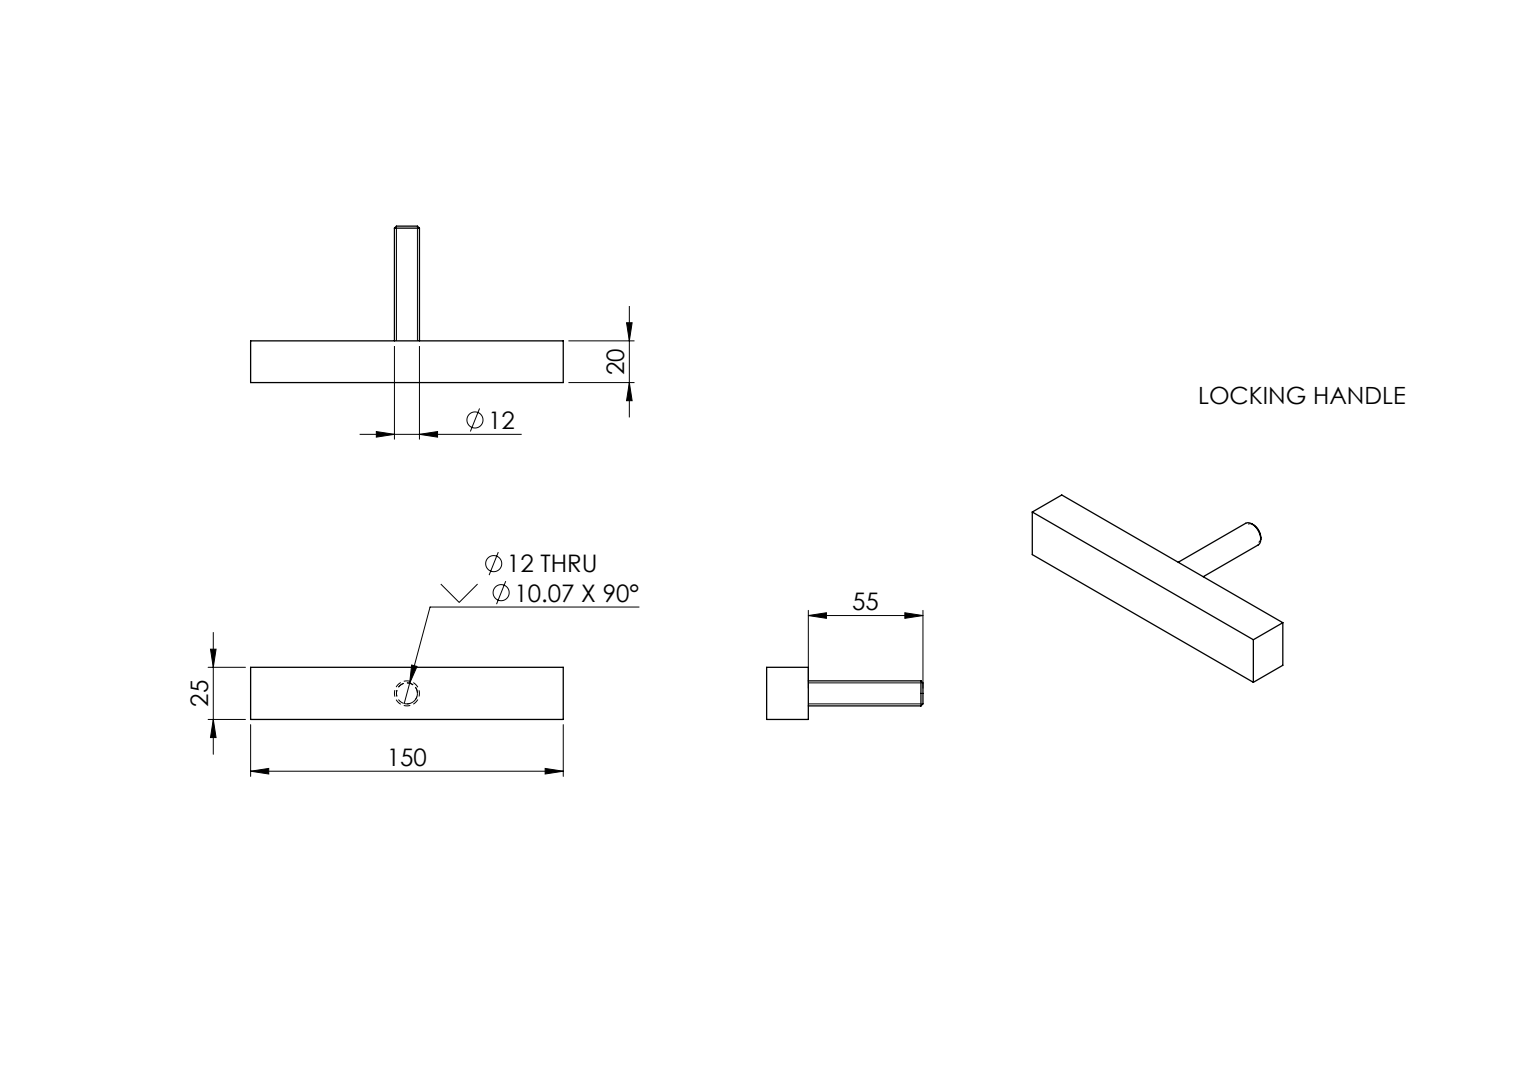
ISO-10303-21;
HEADER;
FILE_DESCRIPTION (('STEP AP214'),
    '1' );
FILE_NAME ('Locking handle.step',
    '2026-10-22T16:49:52',
    ( '' ),
    ( '' ),
    'SwSTEP 2.0',
    'SolidWorks 2026',
    '' );
FILE_SCHEMA (( 'AUTOMOTIVE_DESIGN' ));
ENDSEC;

DATA;
#11=EDGE_CURVE ( 'NONE', #3738, #432, #4098, .T. ) ;
#12=ORIENTED_EDGE ( 'NONE', *, *, #4828, .T. ) ;
#13=DIRECTION ( 'NONE',  ( 7.401486830834378251E-16, -1.000000000000000000, 0.000000000000000000 ) ) ;
#16=EDGE_CURVE ( 'NONE', #5260, #261, #3181, .T. ) ;
#28=EDGE_LOOP ( 'NONE', ( #1037, #4864, #2855, #4479 ) ) ;
#37=CARTESIAN_POINT ( 'NONE',  ( -74.99999999999998579, 610.0000000000000000, 49.99999999999998579 ) ) ;
#52=EDGE_CURVE ( 'NONE', #4486, #4891, #4610, .T. ) ;
#53=EDGE_LOOP ( 'NONE', ( #12, #4860, #912, #4381 ) ) ;
#54=AXIS2_PLACEMENT_3D ( 'NONE', #1971, #1612, #2923 ) ;
#85=FACE_OUTER_BOUND ( 'NONE', #3426, .T. ) ;
#114=DIRECTION ( 'NONE',  ( 1.000000000000000000, 0.000000000000000000, 0.000000000000000000 ) ) ;
#120=EDGE_LOOP ( 'NONE', ( #3988, #3057, #2483, #2092 ) ) ;
#121=SHAPE_REPRESENTATION ( 'Locking handle', ( #4154 ), #2227 ) ;
#140=AXIS2_PLACEMENT_3D ( 'NONE', #4031, #279, #2385 ) ;
#141=COLOUR_RGB ( '',0.8941176470588234615, 0.8941176470588234615, 0.8941176470588234615 ) ;
#146=CARTESIAN_POINT ( 'NONE',  ( -74.99999999999998579, 582.4999999999997726, 49.99999999999998579 ) ) ;
#172=MECHANICAL_DESIGN_GEOMETRIC_PRESENTATION_REPRESENTATION('',(#4869),#4866);
#231=PLANE ( 'NONE',  #3894 ) ;
#258=MANIFOLD_SOLID_BREP ( 'M12 Machine Threads Stud1', #3451 ) ;
#259=ORIENTED_EDGE ( 'NONE', *, *, #2872, .T. ) ;
#261=VERTEX_POINT ( 'NONE', #1126 ) ;
#275=DIRECTION ( 'NONE',  ( 1.000000000000000000, 0.000000000000000000, 0.000000000000000000 ) ) ;
#276=ORIENTED_EDGE ( 'NONE', *, *, #1791, .T. ) ;
#279=DIRECTION ( 'NONE',  ( -0.000000000000000000, -0.000000000000000000, 1.000000000000000000 ) ) ;
#283=DIRECTION ( 'NONE',  ( -0.000000000000000000, -0.000000000000000000, 1.000000000000000000 ) ) ;
#295=AXIS2_PLACEMENT_3D ( 'NONE', #2964, #518, #4278 ) ;
#317=PLANE ( 'NONE',  #5199 ) ;
#334=AXIS2_PLACEMENT_3D ( 'NONE', #394, #283, #1936 ) ;
#343=ORIENTED_EDGE ( 'NONE', *, *, #2742, .T. ) ;
#349=CARTESIAN_POINT ( 'NONE',  ( -1.144917494144692998E-14, 570.0000000000000000, -24.99999999999998579 ) ) ;
#372=ADVANCED_FACE ( 'NONE', ( #4132 ), #2916, .F. ) ;
#373=ORIENTED_EDGE ( 'NONE', *, *, #3431, .F. ) ;
#388=PLANE ( 'NONE',  #3538 ) ;
#390=VECTOR ( 'NONE', #4500, 1000.000000000000000 ) ;
#394=CARTESIAN_POINT ( 'NONE',  ( -1.144917494144692998E-14, 570.0000000000000000, -24.03599999999999071 ) ) ;
#409=ORIENTED_EDGE ( 'NONE', *, *, #3431, .T. ) ;
#432=VERTEX_POINT ( 'NONE', #439 ) ;
#439=CARTESIAN_POINT ( 'NONE',  ( -74.99999999999998579, 582.4999999999997726, 49.99999999999998579 ) ) ;
#458=EDGE_CURVE ( 'NONE', #3578, #4918, #3803, .T. ) ;
#469=SURFACE_STYLE_USAGE ( .BOTH. , #4208 ) ;
#470=EDGE_CURVE ( 'NONE', #4891, #4946, #540, .T. ) ;
#501=APPLICATION_CONTEXT ( 'automotive_design' ) ;
#510=DIRECTION ( 'NONE',  ( -0.000000000000000000, -0.000000000000000000, 1.000000000000000000 ) ) ;
#518=DIRECTION ( 'NONE',  ( 0.000000000000000000, 0.000000000000000000, -1.000000000000000000 ) ) ;
#533=EDGE_CURVE ( 'NONE', #432, #3578, #4203, .T. ) ;
#540=LINE ( 'NONE', #569, #3063 ) ;
#569=CARTESIAN_POINT ( 'NONE',  ( 1.410908427127813464E-14, 582.4999999999997726, 30.00000000000000711 ) ) ;
#581=LINE ( 'NONE', #1466, #1103 ) ;
#594=ORIENTED_EDGE ( 'NONE', *, *, #829, .T. ) ;
#600=DIRECTION ( 'NONE',  ( -0.000000000000000000, -0.000000000000000000, 1.000000000000000000 ) ) ;
#608=ORIENTED_EDGE ( 'NONE', *, *, #458, .F. ) ;
#671=ORIENTED_EDGE ( 'NONE', *, *, #1136, .T. ) ;
#679=AXIS2_PLACEMENT_3D ( 'NONE', #2078, #13, #3676 ) ;
#688=EDGE_CURVE ( 'NONE', #1702, #1418, #2388, .T. ) ;
#729=CARTESIAN_POINT ( 'NONE',  ( 75.00000000000001421, 610.0000000000000000, 30.00000000000002487 ) ) ;
#757=UNCERTAINTY_MEASURE_WITH_UNIT (LENGTH_MEASURE( 1.000000000000000082E-05 ), #1560, 'distance_accuracy_value', 'NONE');
#760=ADVANCED_FACE ( 'NONE', ( #5235 ), #3158, .T. ) ;
#764=ORIENTED_EDGE ( 'NONE', *, *, #1472, .T. ) ;
#769=DIRECTION ( 'NONE',  ( 1.000000000000000000, 0.000000000000000000, 0.000000000000000000 ) ) ;
#805=ORIENTED_EDGE ( 'NONE', *, *, #4792, .T. ) ;
#812=CARTESIAN_POINT ( 'NONE',  ( -1.144917494144692998E-14, 570.0000000000000000, 30.00000000000001066 ) ) ;
#829=EDGE_CURVE ( 'NONE', #3578, #1196, #3313, .T. ) ;
#830=LINE ( 'NONE', #3422, #4489 ) ;
#839=AXIS2_PLACEMENT_3D ( 'NONE', #349, #4430, #864 ) ;
#864=DIRECTION ( 'NONE',  ( 1.000000000000000000, 0.000000000000000000, 0.000000000000000000 ) ) ;
#884=CARTESIAN_POINT ( 'NONE',  ( 5.999999999999983125, 570.0000000000000000, -24.03599999999999071 ) ) ;
#907=CARTESIAN_POINT ( 'NONE',  ( -1.144917494144692998E-14, 570.0000000000000000, 30.00000000000001066 ) ) ;
#909=AXIS2_PLACEMENT_3D ( 'NONE', #907, #510, #3839 ) ;
#912=ORIENTED_EDGE ( 'NONE', *, *, #533, .F. ) ;
#926=DIRECTION ( 'NONE',  ( 1.000000000000000000, 0.000000000000000000, -0.000000000000000000 ) ) ;
#953=CARTESIAN_POINT ( 'NONE',  ( 75.00000000000001421, 610.0000000000000000, 50.00000000000002132 ) ) ;
#965=VECTOR ( 'NONE', #2398, 1000.000000000000000 ) ;
#999=VECTOR ( 'NONE', #3243, 1000.000000000000000 ) ;
#1010=VECTOR ( 'NONE', #1523, 999.9999999999998863 ) ;
#1013=EDGE_LOOP ( 'NONE', ( #4222, #3217 ) ) ;
#1015=CARTESIAN_POINT ( 'NONE',  ( -1.144917494144692998E-14, 570.0000000000000000, -24.03599999999999071 ) ) ;
#1019=DIRECTION ( 'NONE',  ( -0.000000000000000000, -0.000000000000000000, -1.000000000000000000 ) ) ;
#1036=ORIENTED_EDGE ( 'NONE', *, *, #3071, .T. ) ;
#1037=ORIENTED_EDGE ( 'NONE', *, *, #2742, .F. ) ;
#1048=LINE ( 'NONE', #4368, #1525 ) ;
#1092=PRODUCT_DEFINITION_FORMATION_WITH_SPECIFIED_SOURCE ( 'ANY', '', #4530, .NOT_KNOWN. ) ;
#1103=VECTOR ( 'NONE', #2269, 999.9999999999998863 ) ;
#1126=CARTESIAN_POINT ( 'NONE',  ( -5.036000000000011134, 570.0000000000000000, -24.99999999999998579 ) ) ;
#1134=( NAMED_UNIT ( * ) SI_UNIT ( $, .STERADIAN. ) SOLID_ANGLE_UNIT ( ) );
#1136=EDGE_CURVE ( 'NONE', #2556, #2061, #2486, .T. ) ;
#1149=CARTESIAN_POINT ( 'NONE',  ( 75.00000000000000000, 582.4999999999997726, 50.00000000000001421 ) ) ;
#1153=DIRECTION ( 'NONE',  ( -2.081668171172168513E-16, 0.000000000000000000, 1.000000000000000000 ) ) ;
#1196=VERTEX_POINT ( 'NONE', #1862 ) ;
#1223=DIRECTION ( 'NONE',  ( 0.000000000000000000, 0.000000000000000000, 1.000000000000000000 ) ) ;
#1236=CARTESIAN_POINT ( 'NONE',  ( 5.999999999999988454, 570.0000000000000000, 30.00000000000001066 ) ) ;
#1242=PLANE ( 'NONE',  #54 ) ;
#1259=LINE ( 'NONE', #3374, #1983 ) ;
#1260=SHAPE_REPRESENTATION_RELATIONSHIP ( 'NONE' , 'NONE' ,  #121, #2208 ) ;
#1261=CONICAL_SURFACE ( 'NONE', #5087, 5.999999999999993783, 0.7853981633974491672 ) ;
#1300=ADVANCED_FACE ( 'NONE', ( #4202 ), #3875, .T. ) ;
#1308=DIRECTION ( 'NONE',  ( 1.000000000000000000, -0.000000000000000000, 2.081668171172168513E-16 ) ) ;
#1314=ORIENTED_EDGE ( 'NONE', *, *, #1686, .T. ) ;
#1318=FACE_OUTER_BOUND ( 'NONE', #4015, .T. ) ;
#1329=DIRECTION ( 'NONE',  ( -0.000000000000000000, -0.000000000000000000, 1.000000000000000000 ) ) ;
#1353=CARTESIAN_POINT ( 'NONE',  ( 5.035999999999988042, 570.0000000000000000, -24.99999999999998579 ) ) ;
#1381=DIRECTION ( 'NONE',  ( 0.000000000000000000, -1.000000000000000000, 0.000000000000000000 ) ) ;
#1389=ORIENTED_EDGE ( 'NONE', *, *, #1472, .F. ) ;
#1402=CARTESIAN_POINT ( 'NONE',  ( 75.00000000000000000, 582.4999999999997726, 30.00000000000002132 ) ) ;
#1405=FACE_OUTER_BOUND ( 'NONE', #5287, .T. ) ;
#1418=VERTEX_POINT ( 'NONE', #3558 ) ;
#1431=CARTESIAN_POINT ( 'NONE',  ( 75.00000000000000000, 582.4999999999997726, 50.00000000000001421 ) ) ;
#1465=( LENGTH_UNIT ( ) NAMED_UNIT ( * ) SI_UNIT ( .MILLI., .METRE. ) );
#1466=CARTESIAN_POINT ( 'NONE',  ( -6.000000000000005329, 570.0000000000000000, -24.03599999999999071 ) ) ;
#1472=EDGE_CURVE ( 'NONE', #4918, #3738, #3088, .T. ) ;
#1504=CARTESIAN_POINT ( 'NONE',  ( 1.410908427127813464E-14, 582.4999999999997726, 50.00000000000000000 ) ) ;
#1512=DIRECTION ( 'NONE',  ( -0.000000000000000000, -0.000000000000000000, 1.000000000000000000 ) ) ;
#1523=DIRECTION ( 'NONE',  ( 0.7071067811865482389, 0.000000000000000000, 0.7071067811865469066 ) ) ;
#1525=VECTOR ( 'NONE', #2740, 1000.000000000000000 ) ;
#1527=ADVANCED_FACE ( 'NONE', ( #1405 ), #1261, .T. ) ;
#1531=CARTESIAN_POINT ( 'NONE',  ( -6.245004513516506329E-15, 557.4999999999997726, 50.00000000000000000 ) ) ;
#1552=CARTESIAN_POINT ( 'NONE',  ( -1.144917494144692998E-14, 570.0000000000000000, -24.03599999999999071 ) ) ;
#1553=( NAMED_UNIT ( * ) PLANE_ANGLE_UNIT ( ) SI_UNIT ( $, .RADIAN. ) );
#1555=FACE_BOUND ( 'NONE', #1013, .T. ) ;
#1560=( LENGTH_UNIT ( ) NAMED_UNIT ( * ) SI_UNIT ( .MILLI., .METRE. ) );
#1580=EDGE_CURVE ( 'NONE', #3738, #4891, #4131, .T. ) ;
#1612=DIRECTION ( 'NONE',  ( -1.000000000000000000, 5.551115123125753120E-16, 0.000000000000000000 ) ) ;
#1647=FACE_OUTER_BOUND ( 'NONE', #3306, .T. ) ;
#1686=EDGE_CURVE ( 'NONE', #2061, #2556, #4819, .T. ) ;
#1693=SURFACE_STYLE_FILL_AREA ( #3663 ) ;
#1702=VERTEX_POINT ( 'NONE', #1236 ) ;
#1787=( GEOMETRIC_REPRESENTATION_CONTEXT ( 3 ) GLOBAL_UNCERTAINTY_ASSIGNED_CONTEXT ( ( #4190 ) ) GLOBAL_UNIT_ASSIGNED_CONTEXT ( ( #3858, #4097, #4997 ) ) REPRESENTATION_CONTEXT ( 'NONE', 'WORKASPACE' ) );
#1791=EDGE_CURVE ( 'NONE', #2061, #1418, #3073, .T. ) ;
#1844=CARTESIAN_POINT ( 'NONE',  ( 74.99999999999998579, 557.4999999999997726, 50.00000000000002132 ) ) ;
#1862=CARTESIAN_POINT ( 'NONE',  ( -74.99999999999998579, 557.4999999999997726, 29.99999999999999289 ) ) ;
#1910=CARTESIAN_POINT ( 'NONE',  ( 74.99999999999998579, 557.4999999999997726, 30.00000000000002487 ) ) ;
#1923=CARTESIAN_POINT ( 'NONE',  ( -1.144917494144692998E-14, 570.0000000000000000, 30.00000000000001066 ) ) ;
#1936=DIRECTION ( 'NONE',  ( 1.000000000000000000, 0.000000000000000000, 0.000000000000000000 ) ) ;
#1963=( NAMED_UNIT ( * ) SI_UNIT ( $, .STERADIAN. ) SOLID_ANGLE_UNIT ( ) );
#1971=CARTESIAN_POINT ( 'NONE',  ( 75.00000000000001421, 610.0000000000000000, 50.00000000000002132 ) ) ;
#1972=DIRECTION ( 'NONE',  ( 0.000000000000000000, 1.000000000000000000, -0.000000000000000000 ) ) ;
#1983=VECTOR ( 'NONE', #4207, 1000.000000000000000 ) ;
#2022=CARTESIAN_POINT ( 'NONE',  ( -6.245004513516507118E-15, 0.000000000000000000, 30.00000000000001066 ) ) ;
#2032=VECTOR ( 'NONE', #4152, 1000.000000000000000 ) ;
#2057=CIRCLE ( 'NONE', #140, 5.035999999999999588 ) ;
#2061=VERTEX_POINT ( 'NONE', #4174 ) ;
#2068=AXIS2_PLACEMENT_3D ( 'NONE', #812, #4268, #114 ) ;
#2078=CARTESIAN_POINT ( 'NONE',  ( 1.410908427127813464E-14, 582.4999999999997726, 50.00000000000000000 ) ) ;
#2083=ORIENTED_EDGE ( 'NONE', *, *, #4792, .F. ) ;
#2092=ORIENTED_EDGE ( 'NONE', *, *, #1580, .T. ) ;
#2109=ORIENTED_EDGE ( 'NONE', *, *, #2872, .F. ) ;
#2113=AXIS2_PLACEMENT_3D ( 'NONE', #1923, #1512, #4872 ) ;
#2119=AXIS2_PLACEMENT_3D ( 'NONE', #5170, #3491, #2753 ) ;
#2135=ORIENTED_EDGE ( 'NONE', *, *, #52, .T. ) ;
#2163=EDGE_LOOP ( 'NONE', ( #671, #276, #2307, #5328 ) ) ;
#2188=PRODUCT_DEFINITION ( 'UNKNOWN', '', #1092, #5338 ) ;
#2203=DIRECTION ( 'NONE',  ( -1.000000000000000000, -7.401486830834378251E-16, -2.081668171172168513E-16 ) ) ;
#2206=CARTESIAN_POINT ( 'NONE',  ( -74.99999999999998579, 610.0000000000000000, 29.99999999999999289 ) ) ;
#2208=ADVANCED_BREP_SHAPE_REPRESENTATION ( '', ( #258, #4154 ), #2227 ) ;
#2216=LINE ( 'NONE', #146, #3281 ) ;
#2218=ADVANCED_FACE ( 'NONE', ( #1318 ), #4636, .T. ) ;
#2227=( GEOMETRIC_REPRESENTATION_CONTEXT ( 3 ) GLOBAL_UNCERTAINTY_ASSIGNED_CONTEXT ( ( #757 ) ) GLOBAL_UNIT_ASSIGNED_CONTEXT ( ( #1560, #4036, #1134 ) ) REPRESENTATION_CONTEXT ( 'NONE', 'WORKASPACE' ) );
#2229=VECTOR ( 'NONE', #3421, 1000.000000000000000 ) ;
#2258=ORIENTED_EDGE ( 'NONE', *, *, #1580, .F. ) ;
#2269=DIRECTION ( 'NONE',  ( -0.7071067811865482389, 8.659560562354941486E-17, 0.7071067811865469066 ) ) ;
#2307=ORIENTED_EDGE ( 'NONE', *, *, #688, .F. ) ;
#2373=DIRECTION ( 'NONE',  ( -0.000000000000000000, -0.000000000000000000, 1.000000000000000000 ) ) ;
#2385=DIRECTION ( 'NONE',  ( 1.000000000000000000, 0.000000000000000000, 0.000000000000000000 ) ) ;
#2388=CIRCLE ( 'NONE', #2564, 6.000000000000000000 ) ;
#2398=DIRECTION ( 'NONE',  ( 5.551115123125753120E-16, 1.000000000000000000, 1.155557966632335381E-31 ) ) ;
#2430=VECTOR ( 'NONE', #1381, 1000.000000000000000 ) ;
#2434=CARTESIAN_POINT ( 'NONE',  ( 0.000000000000000000, 0.000000000000000000, 0.000000000000000000 ) ) ;
#2437=ADVANCED_FACE ( 'NONE', ( #3660 ), #1242, .F. ) ;
#2483=ORIENTED_EDGE ( 'NONE', *, *, #11, .F. ) ;
#2486=CIRCLE ( 'NONE', #2119, 5.999999999999993783 ) ;
#2550=CARTESIAN_POINT ( 'NONE',  ( -6.245004513516506329E-15, 557.4999999999997726, 50.00000000000000000 ) ) ;
#2556=VERTEX_POINT ( 'NONE', #884 ) ;
#2564=AXIS2_PLACEMENT_3D ( 'NONE', #4336, #2373, #4438 ) ;
#2589=PRODUCT_DEFINITION_SHAPE ( 'NONE', 'NONE',  #2188 ) ;
#2608=DIRECTION ( 'NONE',  ( -0.000000000000000000, 0.000000000000000000, -1.000000000000000000 ) ) ;
#2613=EDGE_CURVE ( 'NONE', #432, #4946, #2216, .T. ) ;
#2640=DIRECTION ( 'NONE',  ( -0.000000000000000000, -0.000000000000000000, 1.000000000000000000 ) ) ;
#2661=AXIS2_PLACEMENT_3D ( 'NONE', #1552, #2854, #4938 ) ;
#2740=DIRECTION ( 'NONE',  ( 1.000000000000000000, -0.000000000000000000, 2.081668171172168513E-16 ) ) ;
#2742=EDGE_CURVE ( 'NONE', #1196, #4486, #1048, .T. ) ;
#2753=DIRECTION ( 'NONE',  ( 1.000000000000000000, 0.000000000000000000, 0.000000000000000000 ) ) ;
#2765=PRODUCT_CONTEXT ( 'NONE', #501, 'mechanical' ) ;
#2833=ORIENTED_EDGE ( 'NONE', *, *, #11, .T. ) ;
#2838=VECTOR ( 'NONE', #2640, 1000.000000000000000 ) ;
#2847=EDGE_CURVE ( 'NONE', #261, #5260, #2057, .T. ) ;
#2854=DIRECTION ( 'NONE',  ( -0.000000000000000000, -0.000000000000000000, 1.000000000000000000 ) ) ;
#2855=ORIENTED_EDGE ( 'NONE', *, *, #470, .F. ) ;
#2858=DIRECTION ( 'NONE',  ( 1.000000000000000000, 0.000000000000000000, 2.081668171172168513E-16 ) ) ;
#2872=EDGE_CURVE ( 'NONE', #5260, #2556, #5275, .T. ) ;
#2878=ORIENTED_EDGE ( 'NONE', *, *, #1136, .F. ) ;
#2897=ADVANCED_FACE ( 'NONE', ( #1555, #5308 ), #388, .F. ) ;
#2916=PLANE ( 'NONE',  #679 ) ;
#2923=DIRECTION ( 'NONE',  ( -5.551115123125753120E-16, -1.000000000000000000, 0.000000000000000000 ) ) ;
#2964=CARTESIAN_POINT ( 'NONE',  ( 5.035999999999988042, 570.0000000000000000, -24.99999999999998579 ) ) ;
#2986=CARTESIAN_POINT ( 'NONE',  ( -74.99999999999998579, 610.0000000000000000, 49.99999999999998579 ) ) ;
#2992=PRESENTATION_STYLE_ASSIGNMENT (( #469 ) ) ;
#3057=ORIENTED_EDGE ( 'NONE', *, *, #2613, .F. ) ;
#3063=VECTOR ( 'NONE', #2203, 1000.000000000000000 ) ;
#3071=EDGE_CURVE ( 'NONE', #2556, #1702, #830, .T. ) ;
#3073=LINE ( 'NONE', #4691, #2838 ) ;
#3088=LINE ( 'NONE', #953, #4562 ) ;
#3120=DIRECTION ( 'NONE',  ( 5.551115123125753120E-16, 1.000000000000000000, 1.155557966632335381E-31 ) ) ;
#3158=CYLINDRICAL_SURFACE ( 'NONE', #2113, 5.999999999999996447 ) ;
#3181=CIRCLE ( 'NONE', #839, 5.035999999999999588 ) ;
#3217=ORIENTED_EDGE ( 'NONE', *, *, #4327, .T. ) ;
#3243=DIRECTION ( 'NONE',  ( -1.000000000000000000, -7.401486830834378251E-16, -2.081668171172168513E-16 ) ) ;
#3281=VECTOR ( 'NONE', #1019, 1000.000000000000000 ) ;
#3306=EDGE_LOOP ( 'NONE', ( #343, #2083, #608, #594 ) ) ;
#3313=LINE ( 'NONE', #5323, #2032 ) ;
#3374=CARTESIAN_POINT ( 'NONE',  ( 74.99999999999998579, 557.4999999999997726, 50.00000000000002132 ) ) ;
#3405=EDGE_LOOP ( 'NONE', ( #2135, #2258, #1389, #805 ) ) ;
#3421=DIRECTION ( 'NONE',  ( 0.000000000000000000, -1.000000000000000000, 0.000000000000000000 ) ) ;
#3422=CARTESIAN_POINT ( 'NONE',  ( 5.999999999999985789, 570.0000000000000000, 30.00000000000001066 ) ) ;
#3426=EDGE_LOOP ( 'NONE', ( #3604, #764, #2833, #4140 ) ) ;
#3431=EDGE_CURVE ( 'NONE', #261, #2061, #581, .T. ) ;
#3443=EDGE_LOOP ( 'NONE', ( #4424, #5015 ) ) ;
#3451=CLOSED_SHELL ( 'NONE', ( #760, #4270, #4206, #2437, #372, #4774, #4100, #2897, #1300, #1527, #2218 ) ) ;
#3491=DIRECTION ( 'NONE',  ( -0.000000000000000000, -0.000000000000000000, 1.000000000000000000 ) ) ;
#3500=ORIENTED_EDGE ( 'NONE', *, *, #16, .T. ) ;
#3522=CARTESIAN_POINT ( 'NONE',  ( -74.99999999999998579, 582.4999999999997726, 29.99999999999999289 ) ) ;
#3538=AXIS2_PLACEMENT_3D ( 'NONE', #2022, #1153, #2858 ) ;
#3558=CARTESIAN_POINT ( 'NONE',  ( -6.000000000000012434, 570.0000000000000000, 30.00000000000001066 ) ) ;
#3568=DIRECTION ( 'NONE',  ( -2.081668171172168513E-16, 0.000000000000000000, 1.000000000000000000 ) ) ;
#3578=VERTEX_POINT ( 'NONE', #5355 ) ;
#3604=ORIENTED_EDGE ( 'NONE', *, *, #458, .T. ) ;
#3624=FILL_AREA_STYLE_COLOUR ( '', #141 ) ;
#3660=FACE_OUTER_BOUND ( 'NONE', #3405, .T. ) ;
#3663=FILL_AREA_STYLE ('',( #3624 ) ) ;
#3676=DIRECTION ( 'NONE',  ( 1.000000000000000000, 7.401486830834378251E-16, 0.000000000000000000 ) ) ;
#3738=VERTEX_POINT ( 'NONE', #1431 ) ;
#3803=LINE ( 'NONE', #2550, #4513 ) ;
#3805=PLANE ( 'NONE',  #4593 ) ;
#3839=DIRECTION ( 'NONE',  ( 1.000000000000000000, 0.000000000000000000, 0.000000000000000000 ) ) ;
#3858=( LENGTH_UNIT ( ) NAMED_UNIT ( * ) SI_UNIT ( .MILLI., .METRE. ) );
#3875=PLANE ( 'NONE',  #295 ) ;
#3894=AXIS2_PLACEMENT_3D ( 'NONE', #5222, #3568, #5164 ) ;
#3908=LINE ( 'NONE', #2206, #2430 ) ;
#3983=ORIENTED_EDGE ( 'NONE', *, *, #2847, .T. ) ;
#3988=ORIENTED_EDGE ( 'NONE', *, *, #470, .T. ) ;
#4015=EDGE_LOOP ( 'NONE', ( #5372, #1314, #1036, #4748 ) ) ;
#4031=CARTESIAN_POINT ( 'NONE',  ( -1.144917494144692998E-14, 570.0000000000000000, -24.99999999999998579 ) ) ;
#4036=( NAMED_UNIT ( * ) PLANE_ANGLE_UNIT ( ) SI_UNIT ( $, .RADIAN. ) );
#4097=( NAMED_UNIT ( * ) PLANE_ANGLE_UNIT ( ) SI_UNIT ( $, .RADIAN. ) );
#4098=LINE ( 'NONE', #1504, #999 ) ;
#4100=ADVANCED_FACE ( 'NONE', ( #85 ), #231, .T. ) ;
#4117=EDGE_LOOP ( 'NONE', ( #3500, #409, #2878, #2109 ) ) ;
#4131=LINE ( 'NONE', #1149, #390 ) ;
#4132=FACE_OUTER_BOUND ( 'NONE', #120, .T. ) ;
#4140=ORIENTED_EDGE ( 'NONE', *, *, #533, .T. ) ;
#4152=DIRECTION ( 'NONE',  ( -0.000000000000000000, -0.000000000000000000, -1.000000000000000000 ) ) ;
#4154=AXIS2_PLACEMENT_3D ( 'NONE', #2434, #5290, #769 ) ;
#4172=CIRCLE ( 'NONE', #2068, 6.000000000000000000 ) ;
#4174=CARTESIAN_POINT ( 'NONE',  ( -6.000000000000005329, 570.0000000000000000, -24.03599999999999071 ) ) ;
#4190=UNCERTAINTY_MEASURE_WITH_UNIT (LENGTH_MEASURE( 1.000000000000000082E-05 ), #3858, 'distance_accuracy_value', 'NONE');
#4202=FACE_OUTER_BOUND ( 'NONE', #3443, .T. ) ;
#4203=LINE ( 'NONE', #2986, #2229 ) ;
#4206=ADVANCED_FACE ( 'NONE', ( #1647 ), #317, .F. ) ;
#4207=DIRECTION ( 'NONE',  ( -0.000000000000000000, -0.000000000000000000, -1.000000000000000000 ) ) ;
#4208=SURFACE_SIDE_STYLE ('',( #1693 ) ) ;
#4222=ORIENTED_EDGE ( 'NONE', *, *, #688, .T. ) ;
#4268=DIRECTION ( 'NONE',  ( -0.000000000000000000, -0.000000000000000000, 1.000000000000000000 ) ) ;
#4270=ADVANCED_FACE ( 'NONE', ( #4890 ), #5114, .T. ) ;
#4278=DIRECTION ( 'NONE',  ( -1.000000000000000000, 0.000000000000000000, -0.000000000000000000 ) ) ;
#4327=EDGE_CURVE ( 'NONE', #1418, #1702, #4172, .T. ) ;
#4336=CARTESIAN_POINT ( 'NONE',  ( -1.144917494144692998E-14, 570.0000000000000000, 30.00000000000001066 ) ) ;
#4368=CARTESIAN_POINT ( 'NONE',  ( -6.245004513516506329E-15, 557.4999999999997726, 30.00000000000000711 ) ) ;
#4381=ORIENTED_EDGE ( 'NONE', *, *, #2613, .T. ) ;
#4424=ORIENTED_EDGE ( 'NONE', *, *, #16, .F. ) ;
#4430=DIRECTION ( 'NONE',  ( -0.000000000000000000, -0.000000000000000000, 1.000000000000000000 ) ) ;
#4438=DIRECTION ( 'NONE',  ( 1.000000000000000000, 0.000000000000000000, 0.000000000000000000 ) ) ;
#4442=UNCERTAINTY_MEASURE_WITH_UNIT (LENGTH_MEASURE( 1.000000000000000082E-05 ), #1465, 'distance_accuracy_value', 'NONE');
#4447=CARTESIAN_POINT ( 'NONE',  ( 5.999999999999983125, 570.0000000000000000, -24.03599999999999071 ) ) ;
#4479=ORIENTED_EDGE ( 'NONE', *, *, #52, .F. ) ;
#4486=VERTEX_POINT ( 'NONE', #1910 ) ;
#4489=VECTOR ( 'NONE', #1329, 1000.000000000000000 ) ;
#4500=DIRECTION ( 'NONE',  ( -0.000000000000000000, -0.000000000000000000, -1.000000000000000000 ) ) ;
#4513=VECTOR ( 'NONE', #1308, 1000.000000000000000 ) ;
#4523=SHAPE_DEFINITION_REPRESENTATION ( #2589, #121 ) ;
#4530=PRODUCT ( 'Locking handle', 'Locking handle', '', ( #2765 ) ) ;
#4562=VECTOR ( 'NONE', #3120, 1000.000000000000000 ) ;
#4593=AXIS2_PLACEMENT_3D ( 'NONE', #37, #926, #2608 ) ;
#4610=LINE ( 'NONE', #729, #965 ) ;
#4636=CYLINDRICAL_SURFACE ( 'NONE', #909, 5.999999999999996447 ) ;
#4653=FACE_OUTER_BOUND ( 'NONE', #53, .T. ) ;
#4669=ORIENTED_EDGE ( 'NONE', *, *, #1686, .F. ) ;
#4691=CARTESIAN_POINT ( 'NONE',  ( -6.000000000000007994, 570.0000000000000000, 30.00000000000001066 ) ) ;
#4748=ORIENTED_EDGE ( 'NONE', *, *, #4327, .F. ) ;
#4774=ADVANCED_FACE ( 'NONE', ( #4653 ), #3805, .F. ) ;
#4792=EDGE_CURVE ( 'NONE', #4918, #4486, #1259, .T. ) ;
#4819=CIRCLE ( 'NONE', #2661, 5.999999999999993783 ) ;
#4828=EDGE_CURVE ( 'NONE', #4946, #1196, #3908, .T. ) ;
#4842=APPLICATION_CONTEXT ( 'automotive_design' ) ;
#4860=ORIENTED_EDGE ( 'NONE', *, *, #829, .F. ) ;
#4864=ORIENTED_EDGE ( 'NONE', *, *, #4828, .F. ) ;
#4866=( GEOMETRIC_REPRESENTATION_CONTEXT ( 3 ) GLOBAL_UNCERTAINTY_ASSIGNED_CONTEXT ( ( #4442 ) ) GLOBAL_UNIT_ASSIGNED_CONTEXT ( ( #1465, #1553, #1963 ) ) REPRESENTATION_CONTEXT ( 'NONE', 'WORKASPACE' ) );
#4869=STYLED_ITEM('',(#5440),#258);
#4872=DIRECTION ( 'NONE',  ( 1.000000000000000000, 0.000000000000000000, 0.000000000000000000 ) ) ;
#4890=FACE_OUTER_BOUND ( 'NONE', #4117, .T. ) ;
#4891=VERTEX_POINT ( 'NONE', #1402 ) ;
#4918=VERTEX_POINT ( 'NONE', #1844 ) ;
#4938=DIRECTION ( 'NONE',  ( 1.000000000000000000, 0.000000000000000000, 0.000000000000000000 ) ) ;
#4946=VERTEX_POINT ( 'NONE', #3522 ) ;
#4997=( NAMED_UNIT ( * ) SI_UNIT ( $, .STERADIAN. ) SOLID_ANGLE_UNIT ( ) );
#5015=ORIENTED_EDGE ( 'NONE', *, *, #2847, .F. ) ;
#5019=STYLED_ITEM ( 'NONE', ( #2992 ), #2208 ) ;
#5087=AXIS2_PLACEMENT_3D ( 'NONE', #1015, #600, #275 ) ;
#5114=CONICAL_SURFACE ( 'NONE', #334, 5.999999999999993783, 0.7853981633974491672 ) ;
#5164=DIRECTION ( 'NONE',  ( 1.000000000000000000, 0.000000000000000000, 2.081668171172168513E-16 ) ) ;
#5170=CARTESIAN_POINT ( 'NONE',  ( -1.144917494144692998E-14, 570.0000000000000000, -24.03599999999999071 ) ) ;
#5199=AXIS2_PLACEMENT_3D ( 'NONE', #1531, #1972, #1223 ) ;
#5222=CARTESIAN_POINT ( 'NONE',  ( -6.245004513516507118E-15, 0.000000000000000000, 50.00000000000000711 ) ) ;
#5235=FACE_OUTER_BOUND ( 'NONE', #2163, .T. ) ;
#5260=VERTEX_POINT ( 'NONE', #1353 ) ;
#5275=LINE ( 'NONE', #4447, #1010 ) ;
#5285=MECHANICAL_DESIGN_GEOMETRIC_PRESENTATION_REPRESENTATION('',(#5019),#1787);
#5287=EDGE_LOOP ( 'NONE', ( #373, #3983, #259, #4669 ) ) ;
#5290=DIRECTION ( 'NONE',  ( 0.000000000000000000, 0.000000000000000000, 1.000000000000000000 ) ) ;
#5308=FACE_OUTER_BOUND ( 'NONE', #28, .T. ) ;
#5323=CARTESIAN_POINT ( 'NONE',  ( -74.99999999999998579, 557.4999999999997726, 49.99999999999998579 ) ) ;
#5328=ORIENTED_EDGE ( 'NONE', *, *, #3071, .F. ) ;
#5338=PRODUCT_DEFINITION_CONTEXT ( 'detailed design', #4842, 'design' ) ;
#5355=CARTESIAN_POINT ( 'NONE',  ( -74.99999999999998579, 557.4999999999997726, 49.99999999999998579 ) ) ;
#5372=ORIENTED_EDGE ( 'NONE', *, *, #1791, .F. ) ;
#5434=COLOUR_RGB('Off White',0.89,0.88,0.83);
#5435=FILL_AREA_STYLE_COLOUR('',#5434);
#5436=FILL_AREA_STYLE('',(#5435));
#5437=SURFACE_STYLE_FILL_AREA(#5436);
#5438=SURFACE_SIDE_STYLE('',(#5437));
#5439=SURFACE_STYLE_USAGE(.BOTH.,#5438);
#5440=PRESENTATION_STYLE_ASSIGNMENT((#5439));
ENDSEC;
END-ISO-10303-21;
